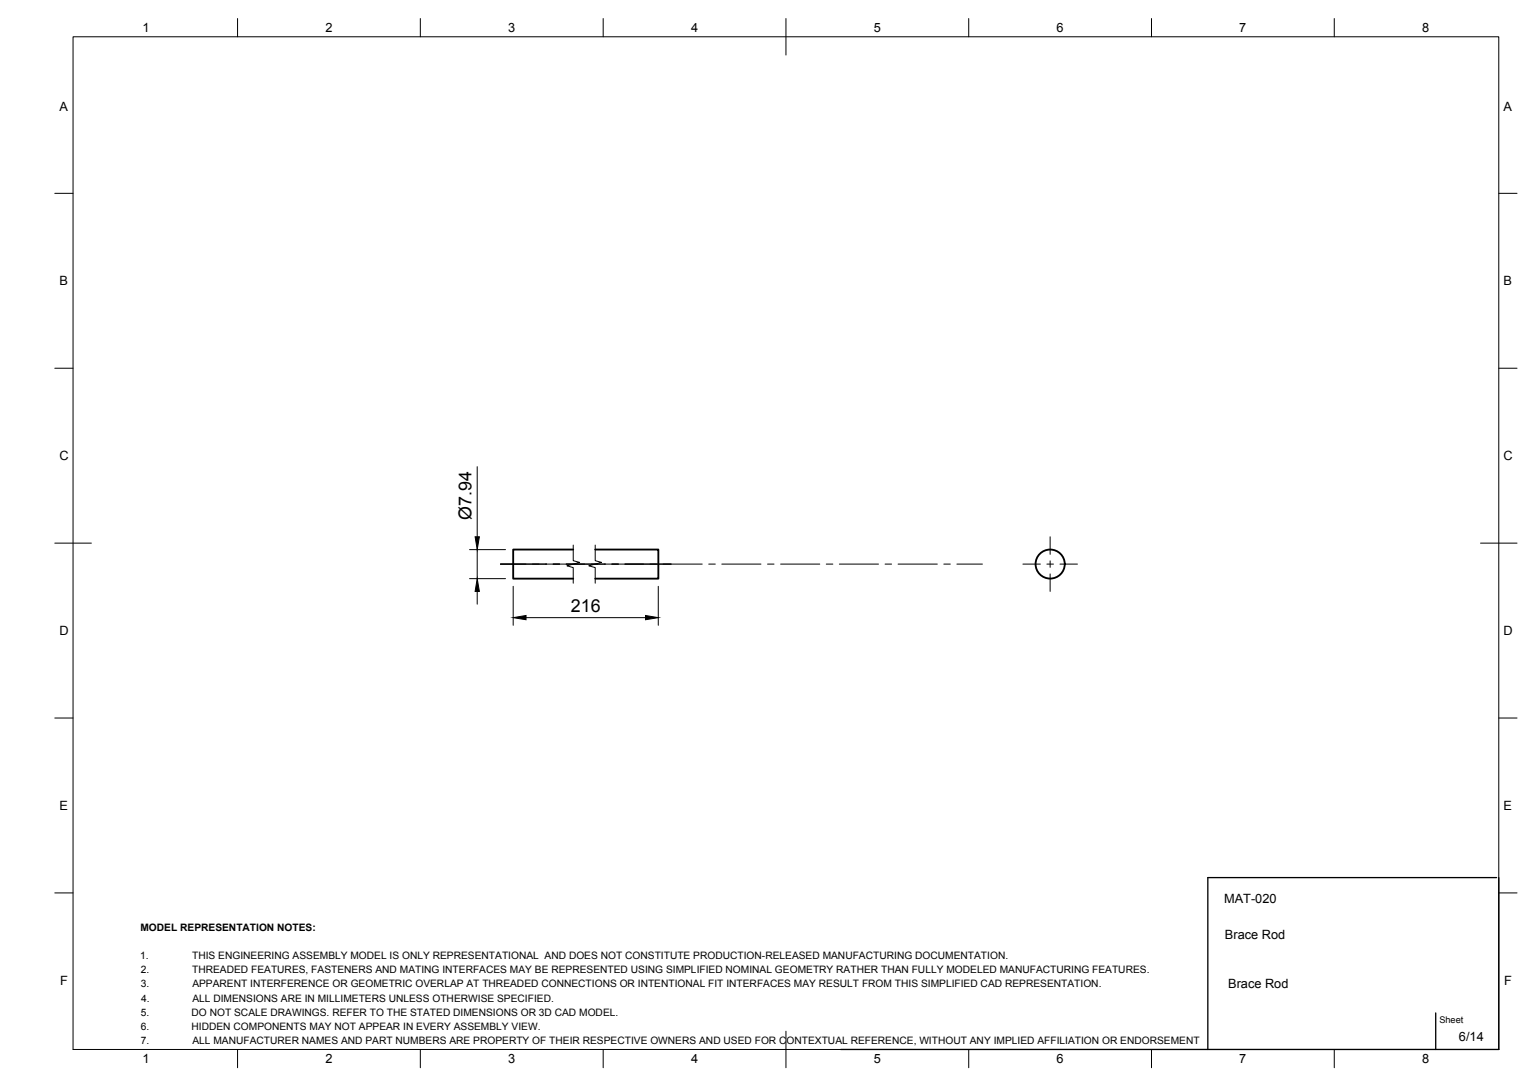
ISO-10303-21;
HEADER;
/* Generated by software containing ST-Developer
 * from STEP Tools, Inc. (www.steptools.com) 
 */

FILE_DESCRIPTION(
/* description */ ('STEP AP214'),
/* implementation_level */ '2;1');

FILE_NAME(
/* name */ 'Brace Rod.step',
/* time_stamp */ '2026-11-14T06:20:50-08:00',
/* author */ (''),
/* organization */ (''),
/* preprocessor_version */ 'ST-DEVELOPER v20.2',
/* originating_system */ 'Autodesk Translation Framework v15.17.0.0',
/* authorisation */ '');

FILE_SCHEMA (('AUTOMOTIVE_DESIGN { 1 0 10303 214 3 1 1 }'));
ENDSEC;

DATA;
#10=MECHANICAL_DESIGN_GEOMETRIC_PRESENTATION_REPRESENTATION('',(#957),#20658);
#393=PLANE('',#3805);
#394=PLANE('',#3806);
#448=LINE('',#4999,#641);
#641=VECTOR('',#4145,3.96875);
#834=CYLINDRICAL_SURFACE('',#3802,3.96875);
#933=SHAPE_REPRESENTATION_RELATIONSHIP('SRR','None',#20717,#945);
#945=ADVANCED_BREP_SHAPE_REPRESENTATION('',(#969),#20647);
#957=STYLED_ITEM('',(#20785),#969);
#969=MANIFOLD_SOLID_BREP('Body1',#3652);
#981=FACE_OUTER_BOUND('',#1190,.T.);
#982=FACE_OUTER_BOUND('',#1191,.T.);
#983=FACE_OUTER_BOUND('',#1192,.T.);
#1190=EDGE_LOOP('',(#2406,#2407,#2408,#2409));
#1191=EDGE_LOOP('',(#2410));
#1192=EDGE_LOOP('',(#2411));
#1423=CIRCLE('',#3803,3.96875);
#1424=CIRCLE('',#3804,3.96875);
#1547=VERTEX_POINT('',#4996);
#1548=VERTEX_POINT('',#4998);
#1885=EDGE_CURVE('',#1547,#1547,#1423,.T.);
#1886=EDGE_CURVE('',#1547,#1548,#448,.T.);
#1887=EDGE_CURVE('',#1548,#1548,#1424,.T.);
#2406=ORIENTED_EDGE('',*,*,#1885,.T.);
#2407=ORIENTED_EDGE('',*,*,#1886,.T.);
#2408=ORIENTED_EDGE('',*,*,#1887,.F.);
#2409=ORIENTED_EDGE('',*,*,#1886,.F.);
#2410=ORIENTED_EDGE('',*,*,#1887,.T.);
#2411=ORIENTED_EDGE('',*,*,#1885,.F.);
#3443=ADVANCED_FACE('',(#981),#834,.T.);
#3444=ADVANCED_FACE('',(#982),#393,.T.);
#3445=ADVANCED_FACE('',(#983),#394,.F.);
#3652=CLOSED_SHELL('',(#3443,#3444,#3445));
#3801=AXIS2_PLACEMENT_3D('',#4994,#4139,#4140);
#3802=AXIS2_PLACEMENT_3D('',#4995,#4141,#4142);
#3803=AXIS2_PLACEMENT_3D('',#4997,#4143,#4144);
#3804=AXIS2_PLACEMENT_3D('',#5000,#4146,#4147);
#3805=AXIS2_PLACEMENT_3D('',#5001,#4148,#4149);
#3806=AXIS2_PLACEMENT_3D('',#5002,#4150,#4151);
#4139=DIRECTION('axis',(0.,0.,1.));
#4140=DIRECTION('refdir',(1.,0.,0.));
#4141=DIRECTION('center_axis',(-1.,0.,0.));
#4142=DIRECTION('ref_axis',(0.,0.,1.));
#4143=DIRECTION('center_axis',(1.,0.,0.));
#4144=DIRECTION('ref_axis',(0.,0.,-1.));
#4145=DIRECTION('',(1.,0.,0.));
#4146=DIRECTION('center_axis',(1.,0.,0.));
#4147=DIRECTION('ref_axis',(0.,0.,-1.));
#4148=DIRECTION('center_axis',(1.,0.,0.));
#4149=DIRECTION('ref_axis',(0.,0.,-1.));
#4150=DIRECTION('center_axis',(1.,0.,0.));
#4151=DIRECTION('ref_axis',(0.,0.,-1.));
#4994=CARTESIAN_POINT('',(0.,0.,0.));
#4995=CARTESIAN_POINT('Origin',(216.,0.,0.));
#4996=CARTESIAN_POINT('',(0.,-4.86031698411606E-16,-3.96875));
#4997=CARTESIAN_POINT('Origin',(0.,0.,0.));
#4998=CARTESIAN_POINT('',(216.,-4.86031698411606E-16,-3.96875));
#4999=CARTESIAN_POINT('',(216.,-4.86031698411606E-16,-3.96875));
#5000=CARTESIAN_POINT('Origin',(216.,0.,0.));
#5001=CARTESIAN_POINT('Origin',(216.,0.,0.));
#5002=CARTESIAN_POINT('Origin',(0.,0.,0.));
#20633=UNCERTAINTY_MEASURE_WITH_UNIT(LENGTH_MEASURE(0.01),#20659,
'DISTANCE_ACCURACY_VALUE',
'Maximum model space distance between geometric entities at asserted c
onnectivities');
#20644=UNCERTAINTY_MEASURE_WITH_UNIT(LENGTH_MEASURE(0.01),#20659,
'DISTANCE_ACCURACY_VALUE',
'Maximum model space distance between geometric entities at asserted c
onnectivities');
#20647=(
GEOMETRIC_REPRESENTATION_CONTEXT(3)
GLOBAL_UNCERTAINTY_ASSIGNED_CONTEXT((#20633))
GLOBAL_UNIT_ASSIGNED_CONTEXT((#20659,#20661,#20662))
REPRESENTATION_CONTEXT('','3D')
);
#20658=(
GEOMETRIC_REPRESENTATION_CONTEXT(3)
GLOBAL_UNCERTAINTY_ASSIGNED_CONTEXT((#20644))
GLOBAL_UNIT_ASSIGNED_CONTEXT((#20659,#20661,#20662))
REPRESENTATION_CONTEXT('','3D')
);
#20659=(
LENGTH_UNIT()
NAMED_UNIT(*)
SI_UNIT(.MILLI.,.METRE.)
);
#20661=(
NAMED_UNIT(*)
PLANE_ANGLE_UNIT()
SI_UNIT($,.RADIAN.)
);
#20662=(
NAMED_UNIT(*)
SI_UNIT($,.STERADIAN.)
SOLID_ANGLE_UNIT()
);
#20665=SHAPE_DEFINITION_REPRESENTATION(#20678,#20717);
#20678=PRODUCT_DEFINITION_SHAPE('',$,#20731);
#20717=SHAPE_REPRESENTATION('',(#3801),#20647);
#20728=PRODUCT_DEFINITION_CONTEXT('part definition',#20769,'design');
#20731=PRODUCT_DEFINITION('Brace Rod','Brace Rod',#20744,#20728);
#20744=PRODUCT_DEFINITION_FORMATION('',$,#20773);
#20769=APPLICATION_CONTEXT(
'Core Data for Automotive Mechanical Design Process');
#20770=PRODUCT_CONTEXT('part definition',#20769,'mechanical');
#20773=PRODUCT('Brace Rod','Brace Rod',$,(#20770));
#20785=PRESENTATION_STYLE_ASSIGNMENT((#20790));
#20790=SURFACE_STYLE_USAGE(.BOTH.,#20795);
#20795=SURFACE_SIDE_STYLE('',(#20800));
#20800=SURFACE_STYLE_FILL_AREA(#20805);
#20805=FILL_AREA_STYLE('Opaque(97,158,199)',(#20810));
#20810=FILL_AREA_STYLE_COLOUR('Opaque(97,158,199)',#20815);
#20815=COLOUR_RGB('Opaque(97,158,199)',0.380392156862745,0.619607843137255,
0.780392156862745);
ENDSEC;
END-ISO-10303-21;
